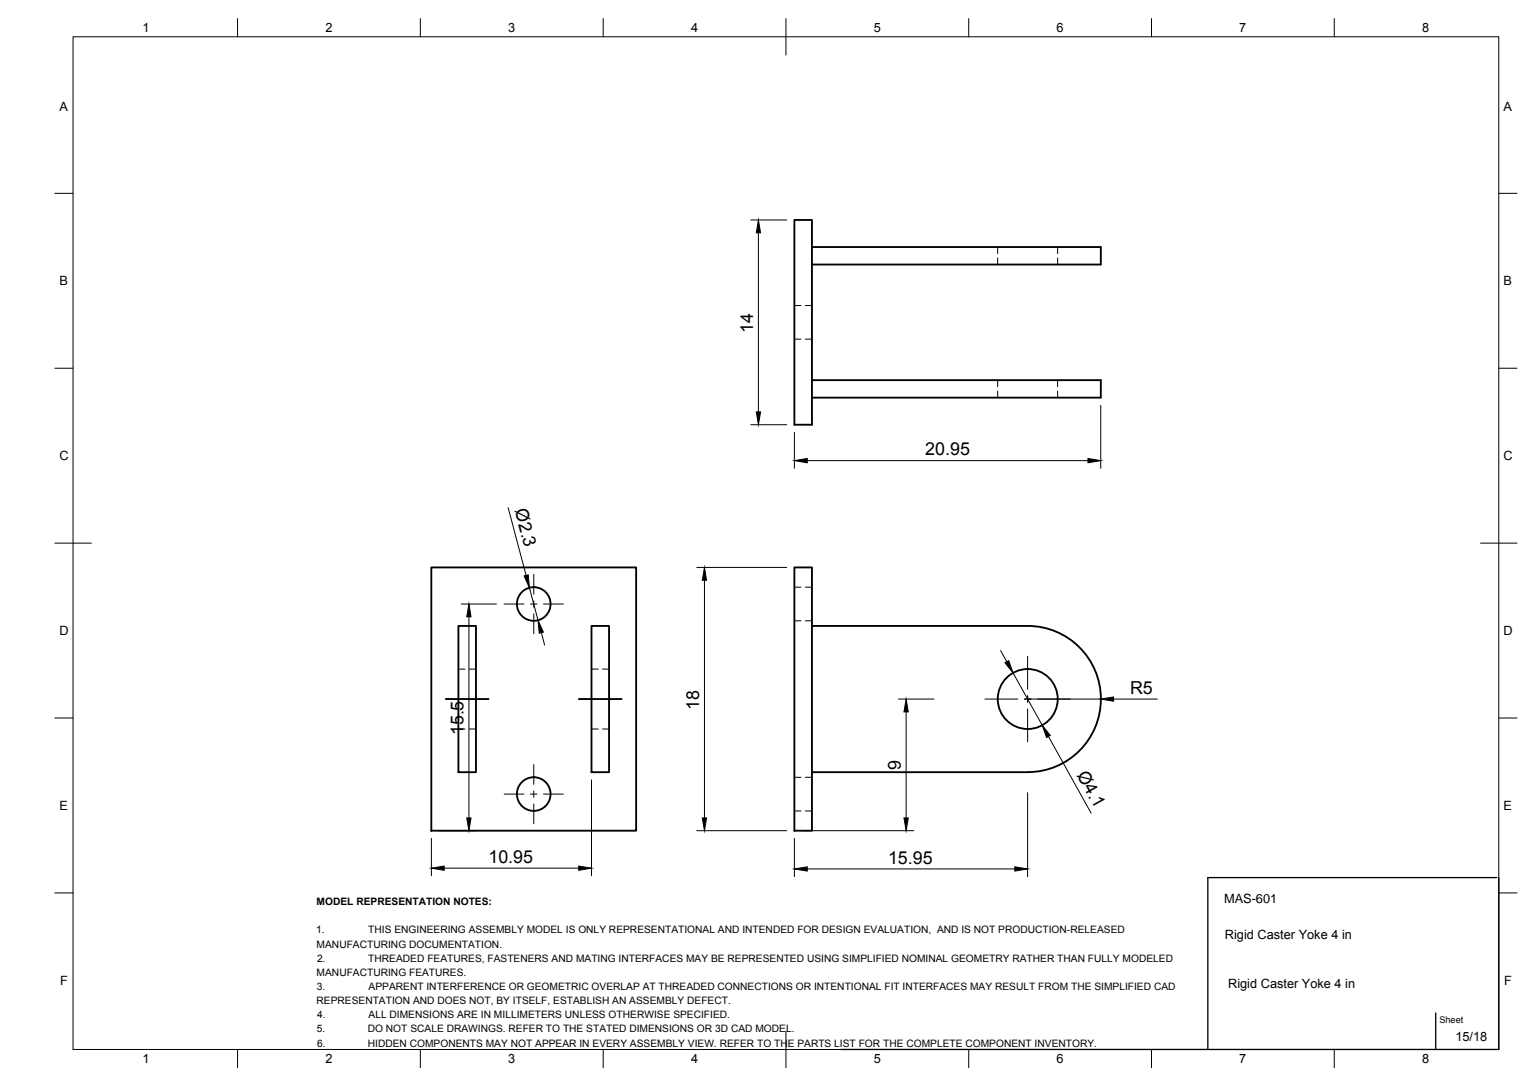
ISO-10303-21;
HEADER;
FILE_DESCRIPTION((''),'2;1');
FILE_NAME('Rigid Caster Yoke 4 in.step','2026-10-06T07:37:42+05:00',(''),(''),'','','');
FILE_SCHEMA (('AUTOMOTIVE_DESIGN { 1 0 10303 214 3 1 1 }'));
ENDSEC;
DATA;
#10=MECHANICAL_DESIGN_GEOMETRIC_PRESENTATION_REPRESENTATION('',(#388),#18757);
#354=SHAPE_REPRESENTATION_RELATIONSHIP('SRR','None',#18872,#371) ;
#371=ADVANCED_BREP_SHAPE_REPRESENTATION('',(#405),#18755) ;
#388=STYLED_ITEM('',(#18966),#405) ;
#405=MANIFOLD_SOLID_BREP('Rigid Caster Yoke 4 in',#9557) ;
#641=CYLINDRICAL_SURFACE('',#10600,1.15) ;
#642=CYLINDRICAL_SURFACE('',#10603,1.15) ;
#643=CYLINDRICAL_SURFACE('',#10610,2.05) ;
#644=CYLINDRICAL_SURFACE('',#10613,4.99999999999999) ;
#645=CYLINDRICAL_SURFACE('',#10620,2.05) ;
#646=CYLINDRICAL_SURFACE('',#10623,4.99999999999999) ;
#745=FACE_BOUND('',#2190,.T.) ;
#746=FACE_BOUND('',#2196,.T.) ;
#747=FACE_BOUND('',#2198,.T.) ;
#748=FACE_BOUND('',#2204,.T.) ;
#749=FACE_BOUND('',#2210,.T.) ;
#750=FACE_BOUND('',#2211,.T.) ;
#751=FACE_BOUND('',#2213,.T.) ;
#752=FACE_BOUND('',#2214,.T.) ;
#753=FACE_BOUND('',#2215,.T.) ;
#754=FACE_BOUND('',#2216,.T.) ;
#1069=PLANE('',#10606) ;
#1070=PLANE('',#10609) ;
#1071=PLANE('',#10612) ;
#1072=PLANE('',#10615) ;
#1073=PLANE('',#10616) ;
#1074=PLANE('',#10619) ;
#1075=PLANE('',#10622) ;
#1076=PLANE('',#10625) ;
#1077=PLANE('',#10626) ;
#1078=PLANE('',#10627) ;
#1079=PLANE('',#10628) ;
#1080=PLANE('',#10629) ;
#1081=PLANE('',#10630) ;
#1082=PLANE('',#10631) ;
#1574=FACE_OUTER_BOUND('',#2187,.T.) ;
#1575=FACE_OUTER_BOUND('',#2188,.T.) ;
#1576=FACE_OUTER_BOUND('',#2189,.T.) ;
#1577=FACE_OUTER_BOUND('',#2191,.T.) ;
#1578=FACE_OUTER_BOUND('',#2192,.T.) ;
#1579=FACE_OUTER_BOUND('',#2193,.T.) ;
#1580=FACE_OUTER_BOUND('',#2194,.T.) ;
#1581=FACE_OUTER_BOUND('',#2195,.T.) ;
#1582=FACE_OUTER_BOUND('',#2197,.T.) ;
#1583=FACE_OUTER_BOUND('',#2199,.T.) ;
#1584=FACE_OUTER_BOUND('',#2200,.T.) ;
#1585=FACE_OUTER_BOUND('',#2201,.T.) ;
#1586=FACE_OUTER_BOUND('',#2202,.T.) ;
#1587=FACE_OUTER_BOUND('',#2203,.T.) ;
#1588=FACE_OUTER_BOUND('',#2205,.T.) ;
#1589=FACE_OUTER_BOUND('',#2206,.T.) ;
#1590=FACE_OUTER_BOUND('',#2207,.T.) ;
#1591=FACE_OUTER_BOUND('',#2208,.T.) ;
#1592=FACE_OUTER_BOUND('',#2209,.T.) ;
#1593=FACE_OUTER_BOUND('',#2212,.T.) ;
#2187=EDGE_LOOP('',(#8857,#8858,#8859,#8860)) ;
#2188=EDGE_LOOP('',(#8861,#8862,#8863,#8864)) ;
#2189=EDGE_LOOP('',(#8865,#8866,#8867,#8868)) ;
#2190=EDGE_LOOP('',(#8869)) ;
#2191=EDGE_LOOP('',(#8870,#8871,#8872,#8873)) ;
#2192=EDGE_LOOP('',(#8874,#8875,#8876,#8877)) ;
#2193=EDGE_LOOP('',(#8878,#8879,#8880,#8881)) ;
#2194=EDGE_LOOP('',(#8882,#8883,#8884,#8885)) ;
#2195=EDGE_LOOP('',(#8886,#8887,#8888,#8889)) ;
#2196=EDGE_LOOP('',(#8890)) ;
#2197=EDGE_LOOP('',(#8891,#8892,#8893,#8894)) ;
#2198=EDGE_LOOP('',(#8895)) ;
#2199=EDGE_LOOP('',(#8896,#8897,#8898,#8899)) ;
#2200=EDGE_LOOP('',(#8900,#8901,#8902,#8903)) ;
#2201=EDGE_LOOP('',(#8904,#8905,#8906,#8907)) ;
#2202=EDGE_LOOP('',(#8908,#8909,#8910,#8911)) ;
#2203=EDGE_LOOP('',(#8912,#8913,#8914,#8915)) ;
#2204=EDGE_LOOP('',(#8916)) ;
#2205=EDGE_LOOP('',(#8917,#8918,#8919,#8920)) ;
#2206=EDGE_LOOP('',(#8921,#8922,#8923,#8924)) ;
#2207=EDGE_LOOP('',(#8925,#8926,#8927,#8928)) ;
#2208=EDGE_LOOP('',(#8929,#8930,#8931,#8932)) ;
#2209=EDGE_LOOP('',(#8933,#8934,#8935,#8936)) ;
#2210=EDGE_LOOP('',(#8937)) ;
#2211=EDGE_LOOP('',(#8938)) ;
#2212=EDGE_LOOP('',(#8939,#8940,#8941,#8942)) ;
#2213=EDGE_LOOP('',(#8943)) ;
#2214=EDGE_LOOP('',(#8944)) ;
#2215=EDGE_LOOP('',(#8945,#8946,#8947,#8948)) ;
#2216=EDGE_LOOP('',(#8949,#8950,#8951,#8952)) ;
#2960=LINE('',#18521,#3731) ;
#2961=LINE('',#18527,#3732) ;
#2962=LINE('',#18532,#3733) ;
#2963=LINE('',#18534,#3734) ;
#2964=LINE('',#18537,#3735) ;
#2965=LINE('',#18542,#3736) ;
#2966=LINE('',#18544,#3737) ;
#2967=LINE('',#18545,#3738) ;
#2968=LINE('',#18548,#3739) ;
#2969=LINE('',#18552,#3740) ;
#2970=LINE('',#18554,#3741) ;
#2971=LINE('',#18555,#3742) ;
#2972=LINE('',#18559,#3743) ;
#2973=LINE('',#18563,#3744) ;
#2974=LINE('',#18565,#3745) ;
#2975=LINE('',#18568,#3746) ;
#2976=LINE('',#18573,#3747) ;
#2977=LINE('',#18575,#3748) ;
#2978=LINE('',#18576,#3749) ;
#2979=LINE('',#18579,#3750) ;
#2980=LINE('',#18583,#3751) ;
#2981=LINE('',#18585,#3752) ;
#2982=LINE('',#18586,#3753) ;
#2983=LINE('',#18590,#3754) ;
#2984=LINE('',#18594,#3755) ;
#2985=LINE('',#18596,#3756) ;
#2986=LINE('',#18598,#3757) ;
#2987=LINE('',#18599,#3758) ;
#2988=LINE('',#18602,#3759) ;
#2989=LINE('',#18604,#3760) ;
#2990=LINE('',#18605,#3761) ;
#2991=LINE('',#18608,#3762) ;
#2992=LINE('',#18610,#3763) ;
#2993=LINE('',#18611,#3764) ;
#2994=LINE('',#18613,#3765) ;
#2995=LINE('',#18614,#3766) ;
#3731=VECTOR('',#13152,1.15) ;
#3732=VECTOR('',#13159,1.15) ;
#3733=VECTOR('',#13164,10.) ;
#3734=VECTOR('',#13165,10.) ;
#3735=VECTOR('',#13168,10.) ;
#3736=VECTOR('',#13173,10.) ;
#3737=VECTOR('',#13174,10.) ;
#3738=VECTOR('',#13175,10.) ;
#3739=VECTOR('',#13178,2.05) ;
#3740=VECTOR('',#13183,10.) ;
#3741=VECTOR('',#13184,10.) ;
#3742=VECTOR('',#13185,10.) ;
#3743=VECTOR('',#13192,10.) ;
#3744=VECTOR('',#13195,10.) ;
#3745=VECTOR('',#13196,10.) ;
#3746=VECTOR('',#13199,10.) ;
#3747=VECTOR('',#13204,10.) ;
#3748=VECTOR('',#13205,10.) ;
#3749=VECTOR('',#13206,10.) ;
#3750=VECTOR('',#13209,2.05) ;
#3751=VECTOR('',#13214,10.) ;
#3752=VECTOR('',#13215,10.) ;
#3753=VECTOR('',#13216,10.) ;
#3754=VECTOR('',#13223,10.) ;
#3755=VECTOR('',#13226,10.) ;
#3756=VECTOR('',#13227,10.) ;
#3757=VECTOR('',#13228,10.) ;
#3758=VECTOR('',#13229,10.) ;
#3759=VECTOR('',#13232,10.) ;
#3760=VECTOR('',#13233,10.) ;
#3761=VECTOR('',#13234,10.) ;
#3762=VECTOR('',#13237,10.) ;
#3763=VECTOR('',#13238,10.) ;
#3764=VECTOR('',#13239,10.) ;
#3765=VECTOR('',#13242,10.) ;
#3766=VECTOR('',#13243,10.) ;
#4126=CIRCLE('',#10601,1.15) ;
#4127=CIRCLE('',#10602,1.15) ;
#4128=CIRCLE('',#10604,1.15) ;
#4129=CIRCLE('',#10605,1.15) ;
#4130=CIRCLE('',#10607,4.99999999999999) ;
#4131=CIRCLE('',#10608,2.05) ;
#4132=CIRCLE('',#10611,2.05) ;
#4133=CIRCLE('',#10614,4.99999999999999) ;
#4134=CIRCLE('',#10617,4.99999999999999) ;
#4135=CIRCLE('',#10618,2.05) ;
#4136=CIRCLE('',#10621,2.05) ;
#4137=CIRCLE('',#10624,4.99999999999999) ;
#4974=VERTEX_POINT('',#18518) ;
#4975=VERTEX_POINT('',#18520) ;
#4976=VERTEX_POINT('',#18524) ;
#4977=VERTEX_POINT('',#18526) ;
#4978=VERTEX_POINT('',#18530) ;
#4979=VERTEX_POINT('',#18531) ;
#4980=VERTEX_POINT('',#18533) ;
#4981=VERTEX_POINT('',#18535) ;
#4982=VERTEX_POINT('',#18538) ;
#4983=VERTEX_POINT('',#18541) ;
#4984=VERTEX_POINT('',#18543) ;
#4985=VERTEX_POINT('',#18547) ;
#4986=VERTEX_POINT('',#18551) ;
#4987=VERTEX_POINT('',#18553) ;
#4988=VERTEX_POINT('',#18561) ;
#4989=VERTEX_POINT('',#18562) ;
#4990=VERTEX_POINT('',#18564) ;
#4991=VERTEX_POINT('',#18566) ;
#4992=VERTEX_POINT('',#18569) ;
#4993=VERTEX_POINT('',#18572) ;
#4994=VERTEX_POINT('',#18574) ;
#4995=VERTEX_POINT('',#18578) ;
#4996=VERTEX_POINT('',#18582) ;
#4997=VERTEX_POINT('',#18584) ;
#4998=VERTEX_POINT('',#18592) ;
#4999=VERTEX_POINT('',#18593) ;
#5000=VERTEX_POINT('',#18595) ;
#5001=VERTEX_POINT('',#18597) ;
#5002=VERTEX_POINT('',#18601) ;
#5003=VERTEX_POINT('',#18603) ;
#5004=VERTEX_POINT('',#18607) ;
#5005=VERTEX_POINT('',#18609) ;
#6275=EDGE_CURVE('',#4974,#4974,#4126,.T.) ;
#6276=EDGE_CURVE('',#4974,#4975,#2960,.T.) ;
#6277=EDGE_CURVE('',#4975,#4975,#4127,.T.) ;
#6278=EDGE_CURVE('',#4976,#4976,#4128,.T.) ;
#6279=EDGE_CURVE('',#4976,#4977,#2961,.T.) ;
#6280=EDGE_CURVE('',#4977,#4977,#4129,.T.) ;
#6281=EDGE_CURVE('',#4978,#4979,#2962,.T.) ;
#6282=EDGE_CURVE('',#4978,#4980,#2963,.T.) ;
#6283=EDGE_CURVE('',#4980,#4981,#4130,.T.) ;
#6284=EDGE_CURVE('',#4981,#4979,#2964,.T.) ;
#6285=EDGE_CURVE('',#4982,#4982,#4131,.T.) ;
#6286=EDGE_CURVE('',#4983,#4978,#2965,.T.) ;
#6287=EDGE_CURVE('',#4983,#4984,#2966,.T.) ;
#6288=EDGE_CURVE('',#4984,#4980,#2967,.T.) ;
#6289=EDGE_CURVE('',#4982,#4985,#2968,.T.) ;
#6290=EDGE_CURVE('',#4985,#4985,#4132,.T.) ;
#6291=EDGE_CURVE('',#4979,#4986,#2969,.T.) ;
#6292=EDGE_CURVE('',#4987,#4981,#2970,.T.) ;
#6293=EDGE_CURVE('',#4987,#4986,#2971,.T.) ;
#6294=EDGE_CURVE('',#4984,#4987,#4133,.T.) ;
#6295=EDGE_CURVE('',#4986,#4983,#2972,.T.) ;
#6296=EDGE_CURVE('',#4988,#4989,#2973,.T.) ;
#6297=EDGE_CURVE('',#4988,#4990,#2974,.T.) ;
#6298=EDGE_CURVE('',#4990,#4991,#4134,.T.) ;
#6299=EDGE_CURVE('',#4991,#4989,#2975,.T.) ;
#6300=EDGE_CURVE('',#4992,#4992,#4135,.T.) ;
#6301=EDGE_CURVE('',#4993,#4988,#2976,.T.) ;
#6302=EDGE_CURVE('',#4993,#4994,#2977,.T.) ;
#6303=EDGE_CURVE('',#4994,#4990,#2978,.T.) ;
#6304=EDGE_CURVE('',#4992,#4995,#2979,.T.) ;
#6305=EDGE_CURVE('',#4995,#4995,#4136,.T.) ;
#6306=EDGE_CURVE('',#4989,#4996,#2980,.T.) ;
#6307=EDGE_CURVE('',#4997,#4991,#2981,.T.) ;
#6308=EDGE_CURVE('',#4997,#4996,#2982,.T.) ;
#6309=EDGE_CURVE('',#4994,#4997,#4137,.T.) ;
#6310=EDGE_CURVE('',#4996,#4993,#2983,.T.) ;
#6311=EDGE_CURVE('',#4998,#4999,#2984,.T.) ;
#6312=EDGE_CURVE('',#4999,#5000,#2985,.T.) ;
#6313=EDGE_CURVE('',#5001,#5000,#2986,.T.) ;
#6314=EDGE_CURVE('',#4998,#5001,#2987,.T.) ;
#6315=EDGE_CURVE('',#5002,#4998,#2988,.T.) ;
#6316=EDGE_CURVE('',#5003,#5001,#2989,.T.) ;
#6317=EDGE_CURVE('',#5002,#5003,#2990,.T.) ;
#6318=EDGE_CURVE('',#5004,#5002,#2991,.T.) ;
#6319=EDGE_CURVE('',#5005,#5003,#2992,.T.) ;
#6320=EDGE_CURVE('',#5004,#5005,#2993,.T.) ;
#6321=EDGE_CURVE('',#4999,#5004,#2994,.T.) ;
#6322=EDGE_CURVE('',#5000,#5005,#2995,.T.) ;
#8857=ORIENTED_EDGE('',*,*,#6275,.F.) ;
#8858=ORIENTED_EDGE('',*,*,#6276,.T.) ;
#8859=ORIENTED_EDGE('',*,*,#6277,.F.) ;
#8860=ORIENTED_EDGE('',*,*,#6276,.F.) ;
#8861=ORIENTED_EDGE('',*,*,#6278,.F.) ;
#8862=ORIENTED_EDGE('',*,*,#6279,.T.) ;
#8863=ORIENTED_EDGE('',*,*,#6280,.F.) ;
#8864=ORIENTED_EDGE('',*,*,#6279,.F.) ;
#8865=ORIENTED_EDGE('',*,*,#6281,.F.) ;
#8866=ORIENTED_EDGE('',*,*,#6282,.T.) ;
#8867=ORIENTED_EDGE('',*,*,#6283,.T.) ;
#8868=ORIENTED_EDGE('',*,*,#6284,.T.) ;
#8869=ORIENTED_EDGE('',*,*,#6285,.T.) ;
#8870=ORIENTED_EDGE('',*,*,#6286,.F.) ;
#8871=ORIENTED_EDGE('',*,*,#6287,.T.) ;
#8872=ORIENTED_EDGE('',*,*,#6288,.T.) ;
#8873=ORIENTED_EDGE('',*,*,#6282,.F.) ;
#8874=ORIENTED_EDGE('',*,*,#6285,.F.) ;
#8875=ORIENTED_EDGE('',*,*,#6289,.T.) ;
#8876=ORIENTED_EDGE('',*,*,#6290,.T.) ;
#8877=ORIENTED_EDGE('',*,*,#6289,.F.) ;
#8878=ORIENTED_EDGE('',*,*,#6291,.F.) ;
#8879=ORIENTED_EDGE('',*,*,#6284,.F.) ;
#8880=ORIENTED_EDGE('',*,*,#6292,.F.) ;
#8881=ORIENTED_EDGE('',*,*,#6293,.T.) ;
#8882=ORIENTED_EDGE('',*,*,#6294,.T.) ;
#8883=ORIENTED_EDGE('',*,*,#6292,.T.) ;
#8884=ORIENTED_EDGE('',*,*,#6283,.F.) ;
#8885=ORIENTED_EDGE('',*,*,#6288,.F.) ;
#8886=ORIENTED_EDGE('',*,*,#6295,.F.) ;
#8887=ORIENTED_EDGE('',*,*,#6293,.F.) ;
#8888=ORIENTED_EDGE('',*,*,#6294,.F.) ;
#8889=ORIENTED_EDGE('',*,*,#6287,.F.) ;
#8890=ORIENTED_EDGE('',*,*,#6290,.F.) ;
#8891=ORIENTED_EDGE('',*,*,#6296,.F.) ;
#8892=ORIENTED_EDGE('',*,*,#6297,.T.) ;
#8893=ORIENTED_EDGE('',*,*,#6298,.T.) ;
#8894=ORIENTED_EDGE('',*,*,#6299,.T.) ;
#8895=ORIENTED_EDGE('',*,*,#6300,.T.) ;
#8896=ORIENTED_EDGE('',*,*,#6301,.F.) ;
#8897=ORIENTED_EDGE('',*,*,#6302,.T.) ;
#8898=ORIENTED_EDGE('',*,*,#6303,.T.) ;
#8899=ORIENTED_EDGE('',*,*,#6297,.F.) ;
#8900=ORIENTED_EDGE('',*,*,#6300,.F.) ;
#8901=ORIENTED_EDGE('',*,*,#6304,.T.) ;
#8902=ORIENTED_EDGE('',*,*,#6305,.T.) ;
#8903=ORIENTED_EDGE('',*,*,#6304,.F.) ;
#8904=ORIENTED_EDGE('',*,*,#6306,.F.) ;
#8905=ORIENTED_EDGE('',*,*,#6299,.F.) ;
#8906=ORIENTED_EDGE('',*,*,#6307,.F.) ;
#8907=ORIENTED_EDGE('',*,*,#6308,.T.) ;
#8908=ORIENTED_EDGE('',*,*,#6309,.T.) ;
#8909=ORIENTED_EDGE('',*,*,#6307,.T.) ;
#8910=ORIENTED_EDGE('',*,*,#6298,.F.) ;
#8911=ORIENTED_EDGE('',*,*,#6303,.F.) ;
#8912=ORIENTED_EDGE('',*,*,#6310,.F.) ;
#8913=ORIENTED_EDGE('',*,*,#6308,.F.) ;
#8914=ORIENTED_EDGE('',*,*,#6309,.F.) ;
#8915=ORIENTED_EDGE('',*,*,#6302,.F.) ;
#8916=ORIENTED_EDGE('',*,*,#6305,.F.) ;
#8917=ORIENTED_EDGE('',*,*,#6311,.T.) ;
#8918=ORIENTED_EDGE('',*,*,#6312,.T.) ;
#8919=ORIENTED_EDGE('',*,*,#6313,.F.) ;
#8920=ORIENTED_EDGE('',*,*,#6314,.F.) ;
#8921=ORIENTED_EDGE('',*,*,#6315,.T.) ;
#8922=ORIENTED_EDGE('',*,*,#6314,.T.) ;
#8923=ORIENTED_EDGE('',*,*,#6316,.F.) ;
#8924=ORIENTED_EDGE('',*,*,#6317,.F.) ;
#8925=ORIENTED_EDGE('',*,*,#6318,.T.) ;
#8926=ORIENTED_EDGE('',*,*,#6317,.T.) ;
#8927=ORIENTED_EDGE('',*,*,#6319,.F.) ;
#8928=ORIENTED_EDGE('',*,*,#6320,.F.) ;
#8929=ORIENTED_EDGE('',*,*,#6321,.T.) ;
#8930=ORIENTED_EDGE('',*,*,#6320,.T.) ;
#8931=ORIENTED_EDGE('',*,*,#6322,.F.) ;
#8932=ORIENTED_EDGE('',*,*,#6312,.F.) ;
#8933=ORIENTED_EDGE('',*,*,#6322,.T.) ;
#8934=ORIENTED_EDGE('',*,*,#6319,.T.) ;
#8935=ORIENTED_EDGE('',*,*,#6316,.T.) ;
#8936=ORIENTED_EDGE('',*,*,#6313,.T.) ;
#8937=ORIENTED_EDGE('',*,*,#6275,.T.) ;
#8938=ORIENTED_EDGE('',*,*,#6278,.T.) ;
#8939=ORIENTED_EDGE('',*,*,#6321,.F.) ;
#8940=ORIENTED_EDGE('',*,*,#6311,.F.) ;
#8941=ORIENTED_EDGE('',*,*,#6315,.F.) ;
#8942=ORIENTED_EDGE('',*,*,#6318,.F.) ;
#8943=ORIENTED_EDGE('',*,*,#6277,.T.) ;
#8944=ORIENTED_EDGE('',*,*,#6280,.T.) ;
#8945=ORIENTED_EDGE('',*,*,#6286,.T.) ;
#8946=ORIENTED_EDGE('',*,*,#6281,.T.) ;
#8947=ORIENTED_EDGE('',*,*,#6291,.T.) ;
#8948=ORIENTED_EDGE('',*,*,#6295,.T.) ;
#8949=ORIENTED_EDGE('',*,*,#6301,.T.) ;
#8950=ORIENTED_EDGE('',*,*,#6296,.T.) ;
#8951=ORIENTED_EDGE('',*,*,#6306,.T.) ;
#8952=ORIENTED_EDGE('',*,*,#6310,.T.) ;
#9510=ADVANCED_FACE('',(#1574),#641,.F.) ;
#9511=ADVANCED_FACE('',(#1575),#642,.F.) ;
#9512=ADVANCED_FACE('',(#1576,#745),#1069,.T.) ;
#9513=ADVANCED_FACE('',(#1577),#1070,.T.) ;
#9514=ADVANCED_FACE('',(#1578),#643,.F.) ;
#9515=ADVANCED_FACE('',(#1579),#1071,.T.) ;
#9516=ADVANCED_FACE('',(#1580),#644,.T.) ;
#9517=ADVANCED_FACE('',(#1581,#746),#1072,.F.) ;
#9518=ADVANCED_FACE('',(#1582,#747),#1073,.T.) ;
#9519=ADVANCED_FACE('',(#1583),#1074,.T.) ;
#9520=ADVANCED_FACE('',(#1584),#645,.F.) ;
#9521=ADVANCED_FACE('',(#1585),#1075,.T.) ;
#9522=ADVANCED_FACE('',(#1586),#646,.T.) ;
#9523=ADVANCED_FACE('',(#1587,#748),#1076,.F.) ;
#9524=ADVANCED_FACE('',(#1588),#1077,.T.) ;
#9525=ADVANCED_FACE('',(#1589),#1078,.T.) ;
#9526=ADVANCED_FACE('',(#1590),#1079,.T.) ;
#9527=ADVANCED_FACE('',(#1591),#1080,.T.) ;
#9528=ADVANCED_FACE('',(#1592,#749,#750),#1081,.T.) ;
#9529=ADVANCED_FACE('',(#1593,#751,#752,#753,#754),#1082,.F.) ;
#9557=CLOSED_SHELL('',(#9510,#9511,#9512,#9513,#9514,#9515,#9516,#9517,
#9518,#9519,#9520,#9521,#9522,#9523,#9524,#9525,#9526,#9527,#9528,#9529)) ;
#10599=AXIS2_PLACEMENT_3D('',#18516,#13146,#13147) ;
#10600=AXIS2_PLACEMENT_3D('',#18517,#13148,#13149) ;
#10601=AXIS2_PLACEMENT_3D('',#18519,#13150,#13151) ;
#10602=AXIS2_PLACEMENT_3D('',#18522,#13153,#13154) ;
#10603=AXIS2_PLACEMENT_3D('',#18523,#13155,#13156) ;
#10604=AXIS2_PLACEMENT_3D('',#18525,#13157,#13158) ;
#10605=AXIS2_PLACEMENT_3D('',#18528,#13160,#13161) ;
#10606=AXIS2_PLACEMENT_3D('',#18529,#13162,#13163) ;
#10607=AXIS2_PLACEMENT_3D('',#18536,#13166,#13167) ;
#10608=AXIS2_PLACEMENT_3D('',#18539,#13169,#13170) ;
#10609=AXIS2_PLACEMENT_3D('',#18540,#13171,#13172) ;
#10610=AXIS2_PLACEMENT_3D('',#18546,#13176,#13177) ;
#10611=AXIS2_PLACEMENT_3D('',#18549,#13179,#13180) ;
#10612=AXIS2_PLACEMENT_3D('',#18550,#13181,#13182) ;
#10613=AXIS2_PLACEMENT_3D('',#18556,#13186,#13187) ;
#10614=AXIS2_PLACEMENT_3D('',#18557,#13188,#13189) ;
#10615=AXIS2_PLACEMENT_3D('',#18558,#13190,#13191) ;
#10616=AXIS2_PLACEMENT_3D('',#18560,#13193,#13194) ;
#10617=AXIS2_PLACEMENT_3D('',#18567,#13197,#13198) ;
#10618=AXIS2_PLACEMENT_3D('',#18570,#13200,#13201) ;
#10619=AXIS2_PLACEMENT_3D('',#18571,#13202,#13203) ;
#10620=AXIS2_PLACEMENT_3D('',#18577,#13207,#13208) ;
#10621=AXIS2_PLACEMENT_3D('',#18580,#13210,#13211) ;
#10622=AXIS2_PLACEMENT_3D('',#18581,#13212,#13213) ;
#10623=AXIS2_PLACEMENT_3D('',#18587,#13217,#13218) ;
#10624=AXIS2_PLACEMENT_3D('',#18588,#13219,#13220) ;
#10625=AXIS2_PLACEMENT_3D('',#18589,#13221,#13222) ;
#10626=AXIS2_PLACEMENT_3D('',#18591,#13224,#13225) ;
#10627=AXIS2_PLACEMENT_3D('',#18600,#13230,#13231) ;
#10628=AXIS2_PLACEMENT_3D('',#18606,#13235,#13236) ;
#10629=AXIS2_PLACEMENT_3D('',#18612,#13240,#13241) ;
#10630=AXIS2_PLACEMENT_3D('',#18615,#13244,#13245) ;
#10631=AXIS2_PLACEMENT_3D('',#18616,#13246,#13247) ;
#13146=DIRECTION('axis',(0.,0.,1.)) ;
#13147=DIRECTION('refdir',(1.,0.,0.)) ;
#13148=DIRECTION('center_axis',(0.,0.,-1.)) ;
#13149=DIRECTION('ref_axis',(1.,0.,0.)) ;
#13150=DIRECTION('center_axis',(0.,0.,-1.)) ;
#13151=DIRECTION('ref_axis',(1.,0.,0.)) ;
#13152=DIRECTION('',(0.,0.,-1.)) ;
#13153=DIRECTION('center_axis',(0.,0.,1.)) ;
#13154=DIRECTION('ref_axis',(1.,0.,0.)) ;
#13155=DIRECTION('center_axis',(0.,0.,-1.)) ;
#13156=DIRECTION('ref_axis',(1.,0.,0.)) ;
#13157=DIRECTION('center_axis',(0.,0.,-1.)) ;
#13158=DIRECTION('ref_axis',(1.,0.,0.)) ;
#13159=DIRECTION('',(0.,0.,-1.)) ;
#13160=DIRECTION('center_axis',(0.,0.,1.)) ;
#13161=DIRECTION('ref_axis',(1.,0.,0.)) ;
#13162=DIRECTION('center_axis',(0.,1.,0.)) ;
#13163=DIRECTION('ref_axis',(1.,0.,0.)) ;
#13164=DIRECTION('',(-1.,0.,0.)) ;
#13165=DIRECTION('',(0.,0.,-1.)) ;
#13166=DIRECTION('center_axis',(0.,1.,0.)) ;
#13167=DIRECTION('ref_axis',(1.,0.,1.33226762955019E-15)) ;
#13168=DIRECTION('',(0.,0.,1.)) ;
#13169=DIRECTION('center_axis',(0.,-1.,0.)) ;
#13170=DIRECTION('ref_axis',(1.,0.,0.)) ;
#13171=DIRECTION('center_axis',(1.,0.,0.)) ;
#13172=DIRECTION('ref_axis',(0.,0.,-1.)) ;
#13173=DIRECTION('',(0.,1.,0.)) ;
#13174=DIRECTION('',(0.,0.,-1.)) ;
#13175=DIRECTION('',(0.,1.,0.)) ;
#13176=DIRECTION('center_axis',(0.,1.,0.)) ;
#13177=DIRECTION('ref_axis',(1.,0.,0.)) ;
#13178=DIRECTION('',(0.,-1.,0.)) ;
#13179=DIRECTION('center_axis',(0.,-1.,0.)) ;
#13180=DIRECTION('ref_axis',(1.,0.,0.)) ;
#13181=DIRECTION('center_axis',(-1.,0.,0.)) ;
#13182=DIRECTION('ref_axis',(0.,0.,1.)) ;
#13183=DIRECTION('',(0.,-1.,0.)) ;
#13184=DIRECTION('',(0.,1.,0.)) ;
#13185=DIRECTION('',(0.,0.,1.)) ;
#13186=DIRECTION('center_axis',(0.,1.,0.)) ;
#13187=DIRECTION('ref_axis',(1.,0.,1.33226762955019E-15)) ;
#13188=DIRECTION('center_axis',(0.,1.,0.)) ;
#13189=DIRECTION('ref_axis',(1.,0.,1.33226762955019E-15)) ;
#13190=DIRECTION('center_axis',(0.,1.,0.)) ;
#13191=DIRECTION('ref_axis',(1.,0.,0.)) ;
#13192=DIRECTION('',(1.,0.,0.)) ;
#13193=DIRECTION('center_axis',(0.,1.,0.)) ;
#13194=DIRECTION('ref_axis',(1.,0.,0.)) ;
#13195=DIRECTION('',(-1.,0.,0.)) ;
#13196=DIRECTION('',(0.,0.,-1.)) ;
#13197=DIRECTION('center_axis',(0.,1.,0.)) ;
#13198=DIRECTION('ref_axis',(1.,0.,1.33226762955019E-15)) ;
#13199=DIRECTION('',(0.,0.,1.)) ;
#13200=DIRECTION('center_axis',(0.,-1.,0.)) ;
#13201=DIRECTION('ref_axis',(1.,0.,0.)) ;
#13202=DIRECTION('center_axis',(1.,0.,0.)) ;
#13203=DIRECTION('ref_axis',(0.,0.,-1.)) ;
#13204=DIRECTION('',(0.,1.,0.)) ;
#13205=DIRECTION('',(0.,0.,-1.)) ;
#13206=DIRECTION('',(0.,1.,0.)) ;
#13207=DIRECTION('center_axis',(0.,1.,0.)) ;
#13208=DIRECTION('ref_axis',(1.,0.,0.)) ;
#13209=DIRECTION('',(0.,-1.,0.)) ;
#13210=DIRECTION('center_axis',(0.,-1.,0.)) ;
#13211=DIRECTION('ref_axis',(1.,0.,0.)) ;
#13212=DIRECTION('center_axis',(-1.,0.,0.)) ;
#13213=DIRECTION('ref_axis',(0.,0.,1.)) ;
#13214=DIRECTION('',(0.,-1.,0.)) ;
#13215=DIRECTION('',(0.,1.,0.)) ;
#13216=DIRECTION('',(0.,0.,1.)) ;
#13217=DIRECTION('center_axis',(0.,1.,0.)) ;
#13218=DIRECTION('ref_axis',(1.,0.,1.33226762955019E-15)) ;
#13219=DIRECTION('center_axis',(0.,1.,0.)) ;
#13220=DIRECTION('ref_axis',(1.,0.,1.33226762955019E-15)) ;
#13221=DIRECTION('center_axis',(0.,1.,0.)) ;
#13222=DIRECTION('ref_axis',(1.,0.,0.)) ;
#13223=DIRECTION('',(1.,0.,0.)) ;
#13224=DIRECTION('center_axis',(0.,1.,0.)) ;
#13225=DIRECTION('ref_axis',(-1.,0.,0.)) ;
#13226=DIRECTION('',(-1.,0.,0.)) ;
#13227=DIRECTION('',(0.,0.,1.)) ;
#13228=DIRECTION('',(-1.,0.,0.)) ;
#13229=DIRECTION('',(0.,0.,1.)) ;
#13230=DIRECTION('center_axis',(1.,0.,0.)) ;
#13231=DIRECTION('ref_axis',(0.,1.,0.)) ;
#13232=DIRECTION('',(0.,1.,0.)) ;
#13233=DIRECTION('',(0.,1.,0.)) ;
#13234=DIRECTION('',(0.,0.,1.)) ;
#13235=DIRECTION('center_axis',(0.,-1.,0.)) ;
#13236=DIRECTION('ref_axis',(1.,0.,0.)) ;
#13237=DIRECTION('',(1.,0.,0.)) ;
#13238=DIRECTION('',(1.,0.,0.)) ;
#13239=DIRECTION('',(0.,0.,1.)) ;
#13240=DIRECTION('center_axis',(-1.,0.,0.)) ;
#13241=DIRECTION('ref_axis',(0.,-1.,0.)) ;
#13242=DIRECTION('',(0.,-1.,0.)) ;
#13243=DIRECTION('',(0.,-1.,0.)) ;
#13244=DIRECTION('center_axis',(0.,0.,1.)) ;
#13245=DIRECTION('ref_axis',(1.,0.,0.)) ;
#13246=DIRECTION('center_axis',(0.,0.,1.)) ;
#13247=DIRECTION('ref_axis',(1.,0.,0.)) ;
#18516=CARTESIAN_POINT('',(0.,0.,0.)) ;
#18517=CARTESIAN_POINT('Origin',(-71.75,52.3,27.6)) ;
#18518=CARTESIAN_POINT('',(-72.9,52.3,27.6)) ;
#18519=CARTESIAN_POINT('Origin',(-71.75,52.3,27.6)) ;
#18520=CARTESIAN_POINT('',(-72.9,52.3,26.4)) ;
#18521=CARTESIAN_POINT('',(-72.9,52.3,27.6)) ;
#18522=CARTESIAN_POINT('Origin',(-71.75,52.3,26.4)) ;
#18523=CARTESIAN_POINT('Origin',(-84.75,52.3,27.6)) ;
#18524=CARTESIAN_POINT('',(-85.9,52.3,27.6)) ;
#18525=CARTESIAN_POINT('Origin',(-84.75,52.3,27.6)) ;
#18526=CARTESIAN_POINT('',(-85.9,52.3,26.4)) ;
#18527=CARTESIAN_POINT('',(-85.9,52.3,27.6)) ;
#18528=CARTESIAN_POINT('Origin',(-84.75,52.3,26.4)) ;
#18529=CARTESIAN_POINT('Origin',(-78.25,48.35,16.775)) ;
#18530=CARTESIAN_POINT('',(-73.25,48.35,26.4)) ;
#18531=CARTESIAN_POINT('',(-83.25,48.35,26.4)) ;
#18532=CARTESIAN_POINT('',(-78.25,48.35,26.4)) ;
#18533=CARTESIAN_POINT('',(-73.25,48.35,11.65)) ;
#18534=CARTESIAN_POINT('',(-73.25,48.35,26.9)) ;
#18535=CARTESIAN_POINT('',(-83.25,48.35,11.65)) ;
#18536=CARTESIAN_POINT('Origin',(-78.25,48.35,11.65)) ;
#18537=CARTESIAN_POINT('',(-83.25,48.35,11.65)) ;
#18538=CARTESIAN_POINT('',(-80.3,48.35,11.65)) ;
#18539=CARTESIAN_POINT('Origin',(-78.25,48.35,11.65)) ;
#18540=CARTESIAN_POINT('Origin',(-73.25,47.15,26.9)) ;
#18541=CARTESIAN_POINT('',(-73.25,47.15,26.4)) ;
#18542=CARTESIAN_POINT('',(-73.25,49.725,26.4)) ;
#18543=CARTESIAN_POINT('',(-73.25,47.15,11.65)) ;
#18544=CARTESIAN_POINT('',(-73.25,47.15,26.9)) ;
#18545=CARTESIAN_POINT('',(-73.25,47.15,11.65)) ;
#18546=CARTESIAN_POINT('Origin',(-78.25,47.15,11.65)) ;
#18547=CARTESIAN_POINT('',(-80.3,47.15,11.65)) ;
#18548=CARTESIAN_POINT('',(-80.3,47.15,11.65)) ;
#18549=CARTESIAN_POINT('Origin',(-78.25,47.15,11.65)) ;
#18550=CARTESIAN_POINT('Origin',(-83.25,47.15,11.65)) ;
#18551=CARTESIAN_POINT('',(-83.25,47.15,26.4)) ;
#18552=CARTESIAN_POINT('',(-83.25,49.725,26.4)) ;
#18553=CARTESIAN_POINT('',(-83.25,47.15,11.65)) ;
#18554=CARTESIAN_POINT('',(-83.25,47.15,11.65)) ;
#18555=CARTESIAN_POINT('',(-83.25,47.15,11.65)) ;
#18556=CARTESIAN_POINT('Origin',(-78.25,47.15,11.65)) ;
#18557=CARTESIAN_POINT('Origin',(-78.25,47.15,11.65)) ;
#18558=CARTESIAN_POINT('Origin',(-78.25,47.15,16.775)) ;
#18559=CARTESIAN_POINT('',(-78.25,47.15,26.4)) ;
#18560=CARTESIAN_POINT('Origin',(-78.25,57.45,16.775)) ;
#18561=CARTESIAN_POINT('',(-73.25,57.45,26.4)) ;
#18562=CARTESIAN_POINT('',(-83.25,57.45,26.4)) ;
#18563=CARTESIAN_POINT('',(-78.25,57.45,26.4)) ;
#18564=CARTESIAN_POINT('',(-73.25,57.45,11.65)) ;
#18565=CARTESIAN_POINT('',(-73.25,57.45,26.9)) ;
#18566=CARTESIAN_POINT('',(-83.25,57.45,11.65)) ;
#18567=CARTESIAN_POINT('Origin',(-78.25,57.45,11.65)) ;
#18568=CARTESIAN_POINT('',(-83.25,57.45,11.65)) ;
#18569=CARTESIAN_POINT('',(-80.3,57.45,11.65)) ;
#18570=CARTESIAN_POINT('Origin',(-78.25,57.45,11.65)) ;
#18571=CARTESIAN_POINT('Origin',(-73.25,56.25,26.9)) ;
#18572=CARTESIAN_POINT('',(-73.25,56.25,26.4)) ;
#18573=CARTESIAN_POINT('',(-73.25,54.275,26.4)) ;
#18574=CARTESIAN_POINT('',(-73.25,56.25,11.65)) ;
#18575=CARTESIAN_POINT('',(-73.25,56.25,26.9)) ;
#18576=CARTESIAN_POINT('',(-73.25,56.25,11.65)) ;
#18577=CARTESIAN_POINT('Origin',(-78.25,56.25,11.65)) ;
#18578=CARTESIAN_POINT('',(-80.3,56.25,11.65)) ;
#18579=CARTESIAN_POINT('',(-80.3,56.25,11.65)) ;
#18580=CARTESIAN_POINT('Origin',(-78.25,56.25,11.65)) ;
#18581=CARTESIAN_POINT('Origin',(-83.25,56.25,11.65)) ;
#18582=CARTESIAN_POINT('',(-83.25,56.25,26.4)) ;
#18583=CARTESIAN_POINT('',(-83.25,54.275,26.4)) ;
#18584=CARTESIAN_POINT('',(-83.25,56.25,11.65)) ;
#18585=CARTESIAN_POINT('',(-83.25,56.25,11.65)) ;
#18586=CARTESIAN_POINT('',(-83.25,56.25,11.65)) ;
#18587=CARTESIAN_POINT('Origin',(-78.25,56.25,11.65)) ;
#18588=CARTESIAN_POINT('Origin',(-78.25,56.25,11.65)) ;
#18589=CARTESIAN_POINT('Origin',(-78.25,56.25,16.775)) ;
#18590=CARTESIAN_POINT('',(-78.25,56.25,26.4)) ;
#18591=CARTESIAN_POINT('Origin',(-69.25,59.3,26.4)) ;
#18592=CARTESIAN_POINT('',(-69.25,59.3,26.4)) ;
#18593=CARTESIAN_POINT('',(-87.25,59.3,26.4)) ;
#18594=CARTESIAN_POINT('',(-69.25,59.3,26.4)) ;
#18595=CARTESIAN_POINT('',(-87.25,59.3,27.6)) ;
#18596=CARTESIAN_POINT('',(-87.25,59.3,26.4)) ;
#18597=CARTESIAN_POINT('',(-69.25,59.3,27.6)) ;
#18598=CARTESIAN_POINT('',(-69.25,59.3,27.6)) ;
#18599=CARTESIAN_POINT('',(-69.25,59.3,26.4)) ;
#18600=CARTESIAN_POINT('Origin',(-69.25,45.3,26.4)) ;
#18601=CARTESIAN_POINT('',(-69.25,45.3,26.4)) ;
#18602=CARTESIAN_POINT('',(-69.25,45.3,26.4)) ;
#18603=CARTESIAN_POINT('',(-69.25,45.3,27.6)) ;
#18604=CARTESIAN_POINT('',(-69.25,45.3,27.6)) ;
#18605=CARTESIAN_POINT('',(-69.25,45.3,26.4)) ;
#18606=CARTESIAN_POINT('Origin',(-87.25,45.3,26.4)) ;
#18607=CARTESIAN_POINT('',(-87.25,45.3,26.4)) ;
#18608=CARTESIAN_POINT('',(-87.25,45.3,26.4)) ;
#18609=CARTESIAN_POINT('',(-87.25,45.3,27.6)) ;
#18610=CARTESIAN_POINT('',(-87.25,45.3,27.6)) ;
#18611=CARTESIAN_POINT('',(-87.25,45.3,26.4)) ;
#18612=CARTESIAN_POINT('Origin',(-87.25,59.3,26.4)) ;
#18613=CARTESIAN_POINT('',(-87.25,59.3,26.4)) ;
#18614=CARTESIAN_POINT('',(-87.25,59.3,27.6)) ;
#18615=CARTESIAN_POINT('Origin',(-78.25,52.3,27.6)) ;
#18616=CARTESIAN_POINT('Origin',(-78.25,52.3,26.4)) ;
#18736=UNCERTAINTY_MEASURE_WITH_UNIT(LENGTH_MEASURE(0.01),#18758,
'DISTANCE_ACCURACY_VALUE',
'Maximum model space distance between geometric entities at asserted c
onnectivities') ;
#18738=UNCERTAINTY_MEASURE_WITH_UNIT(LENGTH_MEASURE(0.01),#18758,
'DISTANCE_ACCURACY_VALUE',
'Maximum model space distance between geometric entities at asserted c
onnectivities') ;
#18755=(
GEOMETRIC_REPRESENTATION_CONTEXT(3)
GLOBAL_UNCERTAINTY_ASSIGNED_CONTEXT((#18736))
GLOBAL_UNIT_ASSIGNED_CONTEXT((#18758,#18760,#18761))
REPRESENTATION_CONTEXT('','3D')
) ;
#18757=(
GEOMETRIC_REPRESENTATION_CONTEXT(3)
GLOBAL_UNCERTAINTY_ASSIGNED_CONTEXT((#18738))
GLOBAL_UNIT_ASSIGNED_CONTEXT((#18758,#18760,#18761))
REPRESENTATION_CONTEXT('','3D')
) ;
#18758=(
LENGTH_UNIT()
NAMED_UNIT(*)
SI_UNIT(.MILLI.,.METRE.)
) ;
#18760=(
NAMED_UNIT(*)
PLANE_ANGLE_UNIT()
SI_UNIT($,.RADIAN.)
) ;
#18761=(
NAMED_UNIT(*)
SI_UNIT($,.STERADIAN.)
SOLID_ANGLE_UNIT()
) ;
#18778=SHAPE_DEFINITION_REPRESENTATION(#18796,#18872) ;
#18796=PRODUCT_DEFINITION_SHAPE('',$,#18891) ;
#18872=SHAPE_REPRESENTATION('',(#10599),#18755) ;
#18874=PRODUCT_DEFINITION_CONTEXT('part definition',#18930,'design') ;
#18891=PRODUCT_DEFINITION('Rigid Caster Yoke 4 in',
'Rigid Caster Yoke 4 in',#18909,#18874) ;
#18909=PRODUCT_DEFINITION_FORMATION('',$,#18948) ;
#18930=APPLICATION_CONTEXT(
'Core Data for Automotive Mechanical Design Process') ;
#18931=PRODUCT_CONTEXT('part definition',#18930,'mechanical') ;
#18948=PRODUCT('Rigid Caster Yoke 4 in','Rigid Caster Yoke 4 in',$,(#18931)) ;
#18966=PRESENTATION_STYLE_ASSIGNMENT((#18984)) ;
#18984=SURFACE_STYLE_USAGE(.BOTH.,#19002) ;
#19002=SURFACE_SIDE_STYLE('',(#19020)) ;
#19020=SURFACE_STYLE_FILL_AREA(#19038) ;
#19038=FILL_AREA_STYLE(
'MAS-253 Metallic Sheet - Rigid Caster Yoke 4 in',(#19056)) ;
#19056=FILL_AREA_STYLE_COLOUR(
'MAS-253 Metallic Sheet - Rigid Caster Yoke 4 in',#19074) ;
#19074=COLOUR_RGB('MAS-253 Metallic Sheet - Rigid Caster Yoke 4 in', 0.72549020, 0.75294118, 0.79215686) ;
ENDSEC;
END-ISO-10303-21;
